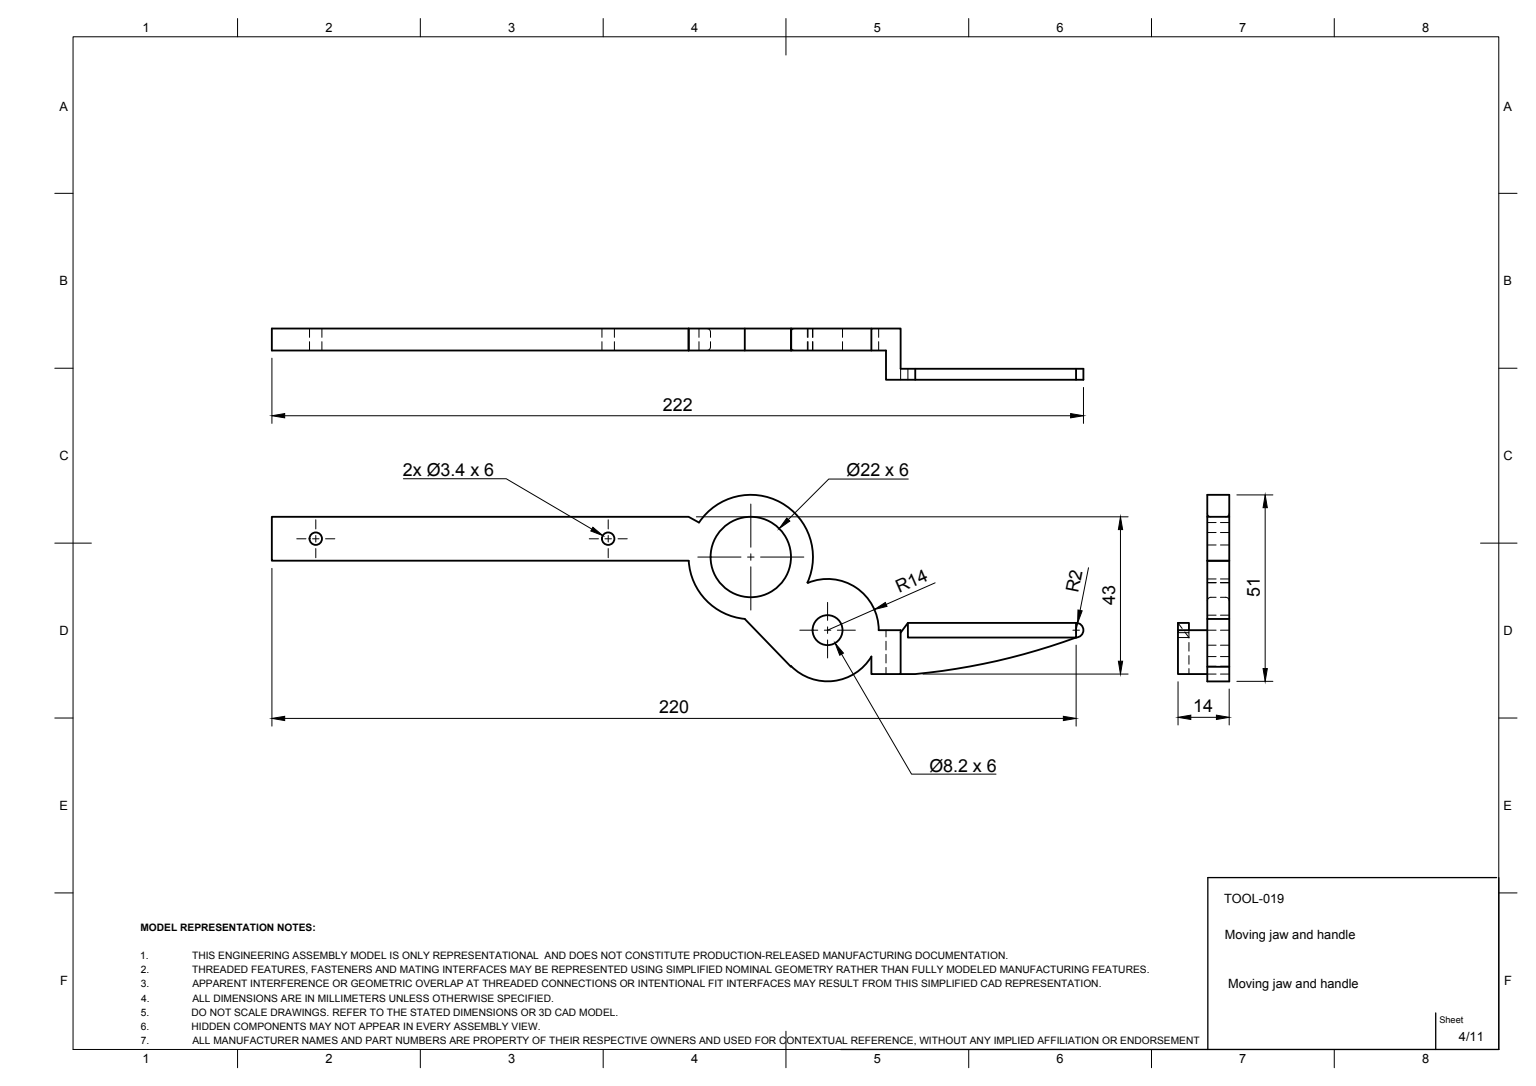
ISO-10303-21;
HEADER;
/* Generated by software containing ST-Developer
 * from STEP Tools, Inc. (www.steptools.com) 
 */

FILE_DESCRIPTION(
/* description */ (''),
/* implementation_level */ '2;1');

FILE_NAME(
/* name */ 'Moving jaw and handle.step',
/* time_stamp */ '2026-11-10T09:14:46-08:00',
/* author */ (''),
/* organization */ (''),
/* preprocessor_version */ 'ST-DEVELOPER v20.2',
/* originating_system */ 'Autodesk Translation Framework v15.17.0.0',
/* authorisation */ '');

FILE_SCHEMA (('AUTOMOTIVE_DESIGN { 1 0 10303 214 3 1 1 }'));
ENDSEC;

DATA;
#10=MECHANICAL_DESIGN_GEOMETRIC_PRESENTATION_REPRESENTATION('',(#559),#19471);
#539=SHAPE_REPRESENTATION_RELATIONSHIP('SRR','None',#19518,#549);
#549=ADVANCED_BREP_SHAPE_REPRESENTATION('',(#569),#19461);
#559=STYLED_ITEM('',(#19581),#569);
#569=MANIFOLD_SOLID_BREP('Body1',#7152);
#580=TOROIDAL_SURFACE('',#7375,1.2,0.1);
#581=TOROIDAL_SURFACE('',#7381,1.2,0.1);
#590=FACE_BOUND('',#1286,.T.);
#591=FACE_BOUND('',#1287,.T.);
#592=FACE_BOUND('',#1288,.T.);
#593=FACE_BOUND('',#1289,.T.);
#594=FACE_BOUND('',#1296,.T.);
#595=FACE_BOUND('',#1297,.T.);
#596=FACE_BOUND('',#1298,.T.);
#597=FACE_BOUND('',#1299,.T.);
#675=PLANE('',#7343);
#676=PLANE('',#7344);
#677=PLANE('',#7345);
#678=PLANE('',#7346);
#679=PLANE('',#7348);
#680=PLANE('',#7350);
#681=PLANE('',#7355);
#682=PLANE('',#7356);
#683=PLANE('',#7357);
#684=PLANE('',#7358);
#685=PLANE('',#7364);
#686=PLANE('',#7365);
#687=PLANE('',#7366);
#688=PLANE('',#7371);
#689=PLANE('',#7385);
#690=PLANE('',#7386);
#691=PLANE('',#7387);
#692=PLANE('',#7388);
#693=PLANE('',#7389);
#694=PLANE('',#7390);
#695=PLANE('',#7391);
#696=PLANE('',#7392);
#854=FACE_OUTER_BOUND('',#1271,.T.);
#855=FACE_OUTER_BOUND('',#1272,.T.);
#856=FACE_OUTER_BOUND('',#1273,.T.);
#857=FACE_OUTER_BOUND('',#1274,.T.);
#858=FACE_OUTER_BOUND('',#1275,.T.);
#859=FACE_OUTER_BOUND('',#1276,.T.);
#860=FACE_OUTER_BOUND('',#1277,.T.);
#861=FACE_OUTER_BOUND('',#1278,.T.);
#862=FACE_OUTER_BOUND('',#1279,.T.);
#863=FACE_OUTER_BOUND('',#1280,.T.);
#864=FACE_OUTER_BOUND('',#1281,.T.);
#865=FACE_OUTER_BOUND('',#1282,.T.);
#866=FACE_OUTER_BOUND('',#1283,.T.);
#867=FACE_OUTER_BOUND('',#1284,.T.);
#868=FACE_OUTER_BOUND('',#1285,.T.);
#869=FACE_OUTER_BOUND('',#1290,.T.);
#870=FACE_OUTER_BOUND('',#1291,.T.);
#871=FACE_OUTER_BOUND('',#1292,.T.);
#872=FACE_OUTER_BOUND('',#1293,.T.);
#873=FACE_OUTER_BOUND('',#1294,.T.);
#874=FACE_OUTER_BOUND('',#1295,.T.);
#875=FACE_OUTER_BOUND('',#1300,.T.);
#876=FACE_OUTER_BOUND('',#1301,.T.);
#877=FACE_OUTER_BOUND('',#1302,.T.);
#878=FACE_OUTER_BOUND('',#1303,.T.);
#879=FACE_OUTER_BOUND('',#1304,.T.);
#880=FACE_OUTER_BOUND('',#1305,.T.);
#881=FACE_OUTER_BOUND('',#1306,.T.);
#882=FACE_OUTER_BOUND('',#1307,.T.);
#883=FACE_OUTER_BOUND('',#1308,.T.);
#884=FACE_OUTER_BOUND('',#1309,.T.);
#885=FACE_OUTER_BOUND('',#1310,.T.);
#886=FACE_OUTER_BOUND('',#1311,.T.);
#887=FACE_OUTER_BOUND('',#1312,.T.);
#1271=EDGE_LOOP('',(#4721,#4722,#4723,#4724));
#1272=EDGE_LOOP('',(#4725,#4726,#4727,#4728));
#1273=EDGE_LOOP('',(#4729,#4730,#4731,#4732));
#1274=EDGE_LOOP('',(#4733,#4734,#4735));
#1275=EDGE_LOOP('',(#4736,#4737,#4738,#4739));
#1276=EDGE_LOOP('',(#4740,#4741,#4742));
#1277=EDGE_LOOP('',(#4743,#4744,#4745,#4746,#4747,#4748));
#1278=EDGE_LOOP('',(#4749,#4750));
#1279=EDGE_LOOP('',(#4751,#4752,#4753,#4754));
#1280=EDGE_LOOP('',(#4755,#4756,#4757,#4758));
#1281=EDGE_LOOP('',(#4759,#4760,#4761,#4762));
#1282=EDGE_LOOP('',(#4763,#4764,#4765,#4766,#4767,#4768,#4769,#4770));
#1283=EDGE_LOOP('',(#4771,#4772,#4773,#4774));
#1284=EDGE_LOOP('',(#4775,#4776,#4777,#4778,#4779,#4780));
#1285=EDGE_LOOP('',(#4781,#4782,#4783,#4784,#4785,#4786,#4787,#4788,#4789,
#4790,#4791,#4792,#4793,#4794,#4795,#4796));
#1286=EDGE_LOOP('',(#4797));
#1287=EDGE_LOOP('',(#4798));
#1288=EDGE_LOOP('',(#4799));
#1289=EDGE_LOOP('',(#4800));
#1290=EDGE_LOOP('',(#4801,#4802,#4803,#4804,#4805,#4806,#4807,#4808));
#1291=EDGE_LOOP('',(#4809,#4810,#4811,#4812,#4813,#4814));
#1292=EDGE_LOOP('',(#4815,#4816,#4817,#4818));
#1293=EDGE_LOOP('',(#4819,#4820,#4821,#4822));
#1294=EDGE_LOOP('',(#4823,#4824,#4825,#4826));
#1295=EDGE_LOOP('',(#4827,#4828,#4829,#4830,#4831,#4832,#4833,#4834,#4835,
#4836,#4837,#4838,#4839,#4840,#4841,#4842));
#1296=EDGE_LOOP('',(#4843));
#1297=EDGE_LOOP('',(#4844));
#1298=EDGE_LOOP('',(#4845));
#1299=EDGE_LOOP('',(#4846));
#1300=EDGE_LOOP('',(#4847,#4848,#4849,#4850));
#1301=EDGE_LOOP('',(#4851,#4852,#4853,#4854,#4855));
#1302=EDGE_LOOP('',(#4856,#4857,#4858,#4859,#4860));
#1303=EDGE_LOOP('',(#4861,#4862,#4863,#4864));
#1304=EDGE_LOOP('',(#4865,#4866,#4867,#4868));
#1305=EDGE_LOOP('',(#4869,#4870,#4871,#4872));
#1306=EDGE_LOOP('',(#4873,#4874,#4875,#4876));
#1307=EDGE_LOOP('',(#4877,#4878,#4879,#4880));
#1308=EDGE_LOOP('',(#4881,#4882,#4883,#4884));
#1309=EDGE_LOOP('',(#4885,#4886,#4887,#4888));
#1310=EDGE_LOOP('',(#4889,#4890,#4891,#4892));
#1311=EDGE_LOOP('',(#4893,#4894,#4895,#4896));
#1312=EDGE_LOOP('',(#4897,#4898,#4899,#4900));
#1774=LINE('',#9576,#2248);
#1775=LINE('',#9582,#2249);
#1776=LINE('',#9588,#2250);
#1777=LINE('',#9593,#2251);
#1778=LINE('',#9595,#2252);
#1779=LINE('',#9596,#2253);
#1780=LINE('',#9600,#2254);
#1781=LINE('',#9601,#2255);
#1782=LINE('',#9602,#2256);
#1783=LINE('',#9605,#2257);
#1784=LINE('',#9606,#2258);
#1785=LINE('',#9609,#2259);
#1786=LINE('',#9611,#2260);
#1787=LINE('',#9613,#2261);
#1788=LINE('',#9619,#2262);
#1789=LINE('',#9620,#2263);
#1790=LINE('',#9624,#2264);
#1791=LINE('',#9628,#2265);
#1792=LINE('',#9632,#2266);
#1793=LINE('',#9634,#2267);
#1794=LINE('',#9635,#2268);
#1795=LINE('',#9636,#2269);
#1796=LINE('',#9639,#2270);
#1797=LINE('',#9641,#2271);
#1798=LINE('',#9642,#2272);
#1799=LINE('',#9645,#2273);
#1800=LINE('',#9647,#2274);
#1801=LINE('',#9649,#2275);
#1802=LINE('',#9650,#2276);
#1803=LINE('',#9653,#2277);
#1804=LINE('',#9655,#2278);
#1805=LINE('',#9659,#2279);
#1806=LINE('',#9661,#2280);
#1807=LINE('',#9665,#2281);
#1808=LINE('',#9667,#2282);
#1809=LINE('',#9669,#2283);
#1810=LINE('',#9671,#2284);
#1811=LINE('',#9673,#2285);
#1812=LINE('',#9677,#2286);
#1813=LINE('',#9683,#2287);
#1814=LINE('',#9685,#2288);
#1815=LINE('',#9686,#2289);
#1816=LINE('',#9688,#2290);
#1817=LINE('',#9691,#2291);
#1818=LINE('',#9692,#2292);
#1819=LINE('',#9695,#2293);
#1820=LINE('',#9700,#2294);
#1821=LINE('',#9703,#2295);
#1822=LINE('',#9707,#2296);
#1823=LINE('',#9709,#2297);
#1824=LINE('',#9711,#2298);
#1825=LINE('',#9713,#2299);
#1826=LINE('',#9715,#2300);
#1827=LINE('',#9719,#2301);
#1828=LINE('',#9720,#2302);
#1829=LINE('',#9732,#2303);
#1830=LINE('',#9736,#2304);
#1831=LINE('',#9737,#2305);
#1832=LINE('',#9739,#2306);
#1833=LINE('',#9740,#2307);
#1834=LINE('',#9742,#2308);
#1835=LINE('',#9744,#2309);
#1836=LINE('',#9747,#2310);
#1837=LINE('',#9750,#2311);
#1838=LINE('',#9752,#2312);
#2248=VECTOR('',#8012,0.17);
#2249=VECTOR('',#8019,0.17);
#2250=VECTOR('',#8026,0.41);
#2251=VECTOR('',#8031,1.);
#2252=VECTOR('',#8032,1.);
#2253=VECTOR('',#8033,1.);
#2254=VECTOR('',#8036,1.);
#2255=VECTOR('',#8037,1.);
#2256=VECTOR('',#8038,1.);
#2257=VECTOR('',#8041,1.);
#2258=VECTOR('',#8042,1.);
#2259=VECTOR('',#8045,1.);
#2260=VECTOR('',#8046,1.);
#2261=VECTOR('',#8047,1.);
#2262=VECTOR('',#8056,1.);
#2263=VECTOR('',#8057,1.);
#2264=VECTOR('',#8062,1.);
#2265=VECTOR('',#8067,1.);
#2266=VECTOR('',#8070,1.);
#2267=VECTOR('',#8071,1.);
#2268=VECTOR('',#8072,1.);
#2269=VECTOR('',#8073,1.);
#2270=VECTOR('',#8076,1.);
#2271=VECTOR('',#8077,1.);
#2272=VECTOR('',#8078,1.);
#2273=VECTOR('',#8081,1.);
#2274=VECTOR('',#8082,1.);
#2275=VECTOR('',#8083,1.);
#2276=VECTOR('',#8084,1.);
#2277=VECTOR('',#8087,1.);
#2278=VECTOR('',#8088,1.);
#2279=VECTOR('',#8091,1.);
#2280=VECTOR('',#8092,1.);
#2281=VECTOR('',#8095,1.);
#2282=VECTOR('',#8096,1.);
#2283=VECTOR('',#8097,1.);
#2284=VECTOR('',#8098,1.);
#2285=VECTOR('',#8099,1.);
#2286=VECTOR('',#8102,1.);
#2287=VECTOR('',#8109,1.);
#2288=VECTOR('',#8110,1.);
#2289=VECTOR('',#8111,1.);
#2290=VECTOR('',#8114,1.);
#2291=VECTOR('',#8117,1.);
#2292=VECTOR('',#8118,1.);
#2293=VECTOR('',#8121,1.);
#2294=VECTOR('',#8128,1.);
#2295=VECTOR('',#8131,1.);
#2296=VECTOR('',#8134,1.);
#2297=VECTOR('',#8135,1.);
#2298=VECTOR('',#8136,1.);
#2299=VECTOR('',#8137,1.);
#2300=VECTOR('',#8138,1.);
#2301=VECTOR('',#8141,1.);
#2302=VECTOR('',#8142,1.);
#2303=VECTOR('',#8157,1.1);
#2304=VECTOR('',#8164,1.);
#2305=VECTOR('',#8165,1.);
#2306=VECTOR('',#8168,1.);
#2307=VECTOR('',#8169,1.);
#2308=VECTOR('',#8172,1.);
#2309=VECTOR('',#8175,1.);
#2310=VECTOR('',#8180,1.);
#2311=VECTOR('',#8185,1.);
#2312=VECTOR('',#8188,1.);
#2682=CIRCLE('',#7335,0.17);
#2683=CIRCLE('',#7336,0.17);
#2684=CIRCLE('',#7338,0.17);
#2685=CIRCLE('',#7339,0.17);
#2686=CIRCLE('',#7341,0.41);
#2687=CIRCLE('',#7342,0.41);
#2688=CIRCLE('',#7347,17.7082646568653);
#2689=CIRCLE('',#7349,0.2);
#2690=CIRCLE('',#7352,0.2);
#2691=CIRCLE('',#7354,17.7082646568653);
#2692=CIRCLE('',#7359,1.4);
#2693=CIRCLE('',#7360,1.7);
#2694=CIRCLE('',#7361,1.7);
#2695=CIRCLE('',#7362,1.4);
#2696=CIRCLE('',#7363,1.2);
#2697=CIRCLE('',#7368,1.4);
#2698=CIRCLE('',#7370,1.4);
#2699=CIRCLE('',#7372,1.7);
#2700=CIRCLE('',#7373,1.7);
#2701=CIRCLE('',#7374,1.2);
#2702=CIRCLE('',#7376,0.1);
#2703=CIRCLE('',#7377,1.1);
#2704=CIRCLE('',#7379,1.1);
#2705=CIRCLE('',#7380,1.1);
#2706=CIRCLE('',#7382,0.1);
#2905=VERTEX_POINT('',#9573);
#2906=VERTEX_POINT('',#9575);
#2907=VERTEX_POINT('',#9579);
#2908=VERTEX_POINT('',#9581);
#2909=VERTEX_POINT('',#9585);
#2910=VERTEX_POINT('',#9587);
#2911=VERTEX_POINT('',#9591);
#2912=VERTEX_POINT('',#9592);
#2913=VERTEX_POINT('',#9594);
#2914=VERTEX_POINT('',#9598);
#2915=VERTEX_POINT('',#9599);
#2916=VERTEX_POINT('',#9604);
#2917=VERTEX_POINT('',#9608);
#2918=VERTEX_POINT('',#9610);
#2919=VERTEX_POINT('',#9612);
#2920=VERTEX_POINT('',#9618);
#2921=VERTEX_POINT('',#9622);
#2922=VERTEX_POINT('',#9626);
#2923=VERTEX_POINT('',#9630);
#2924=VERTEX_POINT('',#9631);
#2925=VERTEX_POINT('',#9633);
#2926=VERTEX_POINT('',#9638);
#2927=VERTEX_POINT('',#9640);
#2928=VERTEX_POINT('',#9644);
#2929=VERTEX_POINT('',#9646);
#2930=VERTEX_POINT('',#9648);
#2931=VERTEX_POINT('',#9652);
#2932=VERTEX_POINT('',#9654);
#2933=VERTEX_POINT('',#9656);
#2934=VERTEX_POINT('',#9658);
#2935=VERTEX_POINT('',#9660);
#2936=VERTEX_POINT('',#9662);
#2937=VERTEX_POINT('',#9664);
#2938=VERTEX_POINT('',#9666);
#2939=VERTEX_POINT('',#9668);
#2940=VERTEX_POINT('',#9670);
#2941=VERTEX_POINT('',#9672);
#2942=VERTEX_POINT('',#9674);
#2943=VERTEX_POINT('',#9676);
#2944=VERTEX_POINT('',#9679);
#2945=VERTEX_POINT('',#9682);
#2946=VERTEX_POINT('',#9684);
#2947=VERTEX_POINT('',#9690);
#2948=VERTEX_POINT('',#9694);
#2949=VERTEX_POINT('',#9698);
#2950=VERTEX_POINT('',#9702);
#2951=VERTEX_POINT('',#9704);
#2952=VERTEX_POINT('',#9706);
#2953=VERTEX_POINT('',#9708);
#2954=VERTEX_POINT('',#9710);
#2955=VERTEX_POINT('',#9712);
#2956=VERTEX_POINT('',#9714);
#2957=VERTEX_POINT('',#9716);
#2958=VERTEX_POINT('',#9718);
#2959=VERTEX_POINT('',#9721);
#2960=VERTEX_POINT('',#9724);
#2961=VERTEX_POINT('',#9728);
#2962=VERTEX_POINT('',#9729);
#3601=EDGE_CURVE('',#2905,#2905,#2682,.T.);
#3602=EDGE_CURVE('',#2905,#2906,#1774,.T.);
#3603=EDGE_CURVE('',#2906,#2906,#2683,.T.);
#3604=EDGE_CURVE('',#2907,#2907,#2684,.T.);
#3605=EDGE_CURVE('',#2907,#2908,#1775,.T.);
#3606=EDGE_CURVE('',#2908,#2908,#2685,.T.);
#3607=EDGE_CURVE('',#2909,#2909,#2686,.T.);
#3608=EDGE_CURVE('',#2909,#2910,#1776,.T.);
#3609=EDGE_CURVE('',#2910,#2910,#2687,.T.);
#3610=EDGE_CURVE('',#2911,#2912,#1777,.T.);
#3611=EDGE_CURVE('',#2913,#2911,#1778,.T.);
#3612=EDGE_CURVE('',#2913,#2912,#1779,.T.);
#3613=EDGE_CURVE('',#2914,#2915,#1780,.T.);
#3614=EDGE_CURVE('',#2913,#2914,#1781,.T.);
#3615=EDGE_CURVE('',#2915,#2911,#1782,.T.);
#3616=EDGE_CURVE('',#2916,#2915,#1783,.T.);
#3617=EDGE_CURVE('',#2914,#2916,#1784,.T.);
#3618=EDGE_CURVE('',#2912,#2917,#1785,.T.);
#3619=EDGE_CURVE('',#2918,#2917,#1786,.T.);
#3620=EDGE_CURVE('',#2918,#2919,#1787,.T.);
#3621=EDGE_CURVE('',#2919,#2915,#2688,.T.);
#3622=EDGE_CURVE('',#2915,#2916,#2689,.T.);
#3623=EDGE_CURVE('',#2917,#2920,#1788,.T.);
#3624=EDGE_CURVE('',#2920,#2913,#1789,.T.);
#3625=EDGE_CURVE('',#2921,#2914,#2690,.T.);
#3626=EDGE_CURVE('',#2921,#2915,#1790,.T.);
#3627=EDGE_CURVE('',#2922,#2921,#2691,.T.);
#3628=EDGE_CURVE('',#2922,#2919,#1791,.T.);
#3629=EDGE_CURVE('',#2923,#2924,#1792,.T.);
#3630=EDGE_CURVE('',#2924,#2925,#1793,.T.);
#3631=EDGE_CURVE('',#2925,#2920,#1794,.T.);
#3632=EDGE_CURVE('',#2922,#2923,#1795,.T.);
#3633=EDGE_CURVE('',#2923,#2926,#1796,.T.);
#3634=EDGE_CURVE('',#2927,#2926,#1797,.T.);
#3635=EDGE_CURVE('',#2924,#2927,#1798,.T.);
#3636=EDGE_CURVE('',#2928,#2927,#1799,.T.);
#3637=EDGE_CURVE('',#2929,#2928,#1800,.T.);
#3638=EDGE_CURVE('',#2930,#2929,#1801,.T.);
#3639=EDGE_CURVE('',#2925,#2930,#1802,.T.);
#3640=EDGE_CURVE('',#2926,#2931,#1803,.T.);
#3641=EDGE_CURVE('',#2931,#2932,#1804,.T.);
#3642=EDGE_CURVE('',#2933,#2932,#2692,.T.);
#3643=EDGE_CURVE('',#2934,#2933,#1805,.T.);
#3644=EDGE_CURVE('',#2935,#2934,#1806,.T.);
#3645=EDGE_CURVE('',#2936,#2935,#2693,.T.);
#3646=EDGE_CURVE('',#2937,#2936,#1807,.T.);
#3647=EDGE_CURVE('',#2938,#2937,#1808,.T.);
#3648=EDGE_CURVE('',#2939,#2938,#1809,.T.);
#3649=EDGE_CURVE('',#2940,#2939,#1810,.T.);
#3650=EDGE_CURVE('',#2941,#2940,#1811,.T.);
#3651=EDGE_CURVE('',#2942,#2941,#2694,.T.);
#3652=EDGE_CURVE('',#2943,#2942,#1812,.T.);
#3653=EDGE_CURVE('',#2928,#2943,#2695,.T.);
#3654=EDGE_CURVE('',#2944,#2944,#2696,.T.);
#3655=EDGE_CURVE('',#2918,#2945,#1813,.T.);
#3656=EDGE_CURVE('',#2946,#2945,#1814,.T.);
#3657=EDGE_CURVE('',#2931,#2946,#1815,.T.);
#3658=EDGE_CURVE('',#2945,#2930,#1816,.T.);
#3659=EDGE_CURVE('',#2932,#2947,#1817,.T.);
#3660=EDGE_CURVE('',#2947,#2946,#1818,.T.);
#3661=EDGE_CURVE('',#2943,#2948,#1819,.T.);
#3662=EDGE_CURVE('',#2929,#2948,#2697,.T.);
#3663=EDGE_CURVE('',#2949,#2947,#2698,.T.);
#3664=EDGE_CURVE('',#2949,#2933,#1820,.T.);
#3665=EDGE_CURVE('',#2948,#2950,#1821,.T.);
#3666=EDGE_CURVE('',#2950,#2951,#2699,.T.);
#3667=EDGE_CURVE('',#2951,#2952,#1822,.T.);
#3668=EDGE_CURVE('',#2952,#2953,#1823,.T.);
#3669=EDGE_CURVE('',#2953,#2954,#1824,.T.);
#3670=EDGE_CURVE('',#2954,#2955,#1825,.T.);
#3671=EDGE_CURVE('',#2955,#2956,#1826,.T.);
#3672=EDGE_CURVE('',#2956,#2957,#2700,.T.);
#3673=EDGE_CURVE('',#2957,#2958,#1827,.T.);
#3674=EDGE_CURVE('',#2958,#2949,#1828,.T.);
#3675=EDGE_CURVE('',#2959,#2959,#2701,.T.);
#3676=EDGE_CURVE('',#2944,#2960,#2702,.T.);
#3677=EDGE_CURVE('',#2960,#2960,#2703,.T.);
#3678=EDGE_CURVE('',#2961,#2962,#2704,.T.);
#3679=EDGE_CURVE('',#2962,#2961,#2705,.T.);
#3680=EDGE_CURVE('',#2962,#2960,#1829,.T.);
#3681=EDGE_CURVE('',#2959,#2961,#2706,.T.);
#3682=EDGE_CURVE('',#2957,#2935,#1830,.T.);
#3683=EDGE_CURVE('',#2936,#2956,#1831,.T.);
#3684=EDGE_CURVE('',#2942,#2950,#1832,.T.);
#3685=EDGE_CURVE('',#2951,#2941,#1833,.T.);
#3686=EDGE_CURVE('',#2940,#2952,#1834,.T.);
#3687=EDGE_CURVE('',#2937,#2955,#1835,.T.);
#3688=EDGE_CURVE('',#2934,#2958,#1836,.T.);
#3689=EDGE_CURVE('',#2938,#2954,#1837,.T.);
#3690=EDGE_CURVE('',#2939,#2953,#1838,.T.);
#4721=ORIENTED_EDGE('',*,*,#3601,.F.);
#4722=ORIENTED_EDGE('',*,*,#3602,.T.);
#4723=ORIENTED_EDGE('',*,*,#3603,.F.);
#4724=ORIENTED_EDGE('',*,*,#3602,.F.);
#4725=ORIENTED_EDGE('',*,*,#3604,.F.);
#4726=ORIENTED_EDGE('',*,*,#3605,.T.);
#4727=ORIENTED_EDGE('',*,*,#3606,.F.);
#4728=ORIENTED_EDGE('',*,*,#3605,.F.);
#4729=ORIENTED_EDGE('',*,*,#3607,.F.);
#4730=ORIENTED_EDGE('',*,*,#3608,.T.);
#4731=ORIENTED_EDGE('',*,*,#3609,.F.);
#4732=ORIENTED_EDGE('',*,*,#3608,.F.);
#4733=ORIENTED_EDGE('',*,*,#3610,.F.);
#4734=ORIENTED_EDGE('',*,*,#3611,.F.);
#4735=ORIENTED_EDGE('',*,*,#3612,.T.);
#4736=ORIENTED_EDGE('',*,*,#3613,.F.);
#4737=ORIENTED_EDGE('',*,*,#3614,.F.);
#4738=ORIENTED_EDGE('',*,*,#3611,.T.);
#4739=ORIENTED_EDGE('',*,*,#3615,.F.);
#4740=ORIENTED_EDGE('',*,*,#3616,.F.);
#4741=ORIENTED_EDGE('',*,*,#3617,.F.);
#4742=ORIENTED_EDGE('',*,*,#3613,.T.);
#4743=ORIENTED_EDGE('',*,*,#3615,.T.);
#4744=ORIENTED_EDGE('',*,*,#3610,.T.);
#4745=ORIENTED_EDGE('',*,*,#3618,.T.);
#4746=ORIENTED_EDGE('',*,*,#3619,.F.);
#4747=ORIENTED_EDGE('',*,*,#3620,.T.);
#4748=ORIENTED_EDGE('',*,*,#3621,.T.);
#4749=ORIENTED_EDGE('',*,*,#3616,.T.);
#4750=ORIENTED_EDGE('',*,*,#3622,.T.);
#4751=ORIENTED_EDGE('',*,*,#3623,.F.);
#4752=ORIENTED_EDGE('',*,*,#3618,.F.);
#4753=ORIENTED_EDGE('',*,*,#3612,.F.);
#4754=ORIENTED_EDGE('',*,*,#3624,.F.);
#4755=ORIENTED_EDGE('',*,*,#3625,.T.);
#4756=ORIENTED_EDGE('',*,*,#3617,.T.);
#4757=ORIENTED_EDGE('',*,*,#3622,.F.);
#4758=ORIENTED_EDGE('',*,*,#3626,.F.);
#4759=ORIENTED_EDGE('',*,*,#3627,.T.);
#4760=ORIENTED_EDGE('',*,*,#3626,.T.);
#4761=ORIENTED_EDGE('',*,*,#3621,.F.);
#4762=ORIENTED_EDGE('',*,*,#3628,.F.);
#4763=ORIENTED_EDGE('',*,*,#3629,.T.);
#4764=ORIENTED_EDGE('',*,*,#3630,.T.);
#4765=ORIENTED_EDGE('',*,*,#3631,.T.);
#4766=ORIENTED_EDGE('',*,*,#3624,.T.);
#4767=ORIENTED_EDGE('',*,*,#3614,.T.);
#4768=ORIENTED_EDGE('',*,*,#3625,.F.);
#4769=ORIENTED_EDGE('',*,*,#3627,.F.);
#4770=ORIENTED_EDGE('',*,*,#3632,.T.);
#4771=ORIENTED_EDGE('',*,*,#3629,.F.);
#4772=ORIENTED_EDGE('',*,*,#3633,.T.);
#4773=ORIENTED_EDGE('',*,*,#3634,.F.);
#4774=ORIENTED_EDGE('',*,*,#3635,.F.);
#4775=ORIENTED_EDGE('',*,*,#3636,.F.);
#4776=ORIENTED_EDGE('',*,*,#3637,.F.);
#4777=ORIENTED_EDGE('',*,*,#3638,.F.);
#4778=ORIENTED_EDGE('',*,*,#3639,.F.);
#4779=ORIENTED_EDGE('',*,*,#3630,.F.);
#4780=ORIENTED_EDGE('',*,*,#3635,.T.);
#4781=ORIENTED_EDGE('',*,*,#3634,.T.);
#4782=ORIENTED_EDGE('',*,*,#3640,.T.);
#4783=ORIENTED_EDGE('',*,*,#3641,.T.);
#4784=ORIENTED_EDGE('',*,*,#3642,.F.);
#4785=ORIENTED_EDGE('',*,*,#3643,.F.);
#4786=ORIENTED_EDGE('',*,*,#3644,.F.);
#4787=ORIENTED_EDGE('',*,*,#3645,.F.);
#4788=ORIENTED_EDGE('',*,*,#3646,.F.);
#4789=ORIENTED_EDGE('',*,*,#3647,.F.);
#4790=ORIENTED_EDGE('',*,*,#3648,.F.);
#4791=ORIENTED_EDGE('',*,*,#3649,.F.);
#4792=ORIENTED_EDGE('',*,*,#3650,.F.);
#4793=ORIENTED_EDGE('',*,*,#3651,.F.);
#4794=ORIENTED_EDGE('',*,*,#3652,.F.);
#4795=ORIENTED_EDGE('',*,*,#3653,.F.);
#4796=ORIENTED_EDGE('',*,*,#3636,.T.);
#4797=ORIENTED_EDGE('',*,*,#3603,.T.);
#4798=ORIENTED_EDGE('',*,*,#3606,.T.);
#4799=ORIENTED_EDGE('',*,*,#3609,.T.);
#4800=ORIENTED_EDGE('',*,*,#3654,.F.);
#4801=ORIENTED_EDGE('',*,*,#3655,.T.);
#4802=ORIENTED_EDGE('',*,*,#3656,.F.);
#4803=ORIENTED_EDGE('',*,*,#3657,.F.);
#4804=ORIENTED_EDGE('',*,*,#3640,.F.);
#4805=ORIENTED_EDGE('',*,*,#3633,.F.);
#4806=ORIENTED_EDGE('',*,*,#3632,.F.);
#4807=ORIENTED_EDGE('',*,*,#3628,.T.);
#4808=ORIENTED_EDGE('',*,*,#3620,.F.);
#4809=ORIENTED_EDGE('',*,*,#3623,.T.);
#4810=ORIENTED_EDGE('',*,*,#3631,.F.);
#4811=ORIENTED_EDGE('',*,*,#3639,.T.);
#4812=ORIENTED_EDGE('',*,*,#3658,.F.);
#4813=ORIENTED_EDGE('',*,*,#3655,.F.);
#4814=ORIENTED_EDGE('',*,*,#3619,.T.);
#4815=ORIENTED_EDGE('',*,*,#3659,.F.);
#4816=ORIENTED_EDGE('',*,*,#3641,.F.);
#4817=ORIENTED_EDGE('',*,*,#3657,.T.);
#4818=ORIENTED_EDGE('',*,*,#3660,.F.);
#4819=ORIENTED_EDGE('',*,*,#3637,.T.);
#4820=ORIENTED_EDGE('',*,*,#3653,.T.);
#4821=ORIENTED_EDGE('',*,*,#3661,.T.);
#4822=ORIENTED_EDGE('',*,*,#3662,.F.);
#4823=ORIENTED_EDGE('',*,*,#3659,.T.);
#4824=ORIENTED_EDGE('',*,*,#3663,.F.);
#4825=ORIENTED_EDGE('',*,*,#3664,.T.);
#4826=ORIENTED_EDGE('',*,*,#3642,.T.);
#4827=ORIENTED_EDGE('',*,*,#3638,.T.);
#4828=ORIENTED_EDGE('',*,*,#3662,.T.);
#4829=ORIENTED_EDGE('',*,*,#3665,.T.);
#4830=ORIENTED_EDGE('',*,*,#3666,.T.);
#4831=ORIENTED_EDGE('',*,*,#3667,.T.);
#4832=ORIENTED_EDGE('',*,*,#3668,.T.);
#4833=ORIENTED_EDGE('',*,*,#3669,.T.);
#4834=ORIENTED_EDGE('',*,*,#3670,.T.);
#4835=ORIENTED_EDGE('',*,*,#3671,.T.);
#4836=ORIENTED_EDGE('',*,*,#3672,.T.);
#4837=ORIENTED_EDGE('',*,*,#3673,.T.);
#4838=ORIENTED_EDGE('',*,*,#3674,.T.);
#4839=ORIENTED_EDGE('',*,*,#3663,.T.);
#4840=ORIENTED_EDGE('',*,*,#3660,.T.);
#4841=ORIENTED_EDGE('',*,*,#3656,.T.);
#4842=ORIENTED_EDGE('',*,*,#3658,.T.);
#4843=ORIENTED_EDGE('',*,*,#3601,.T.);
#4844=ORIENTED_EDGE('',*,*,#3604,.T.);
#4845=ORIENTED_EDGE('',*,*,#3607,.T.);
#4846=ORIENTED_EDGE('',*,*,#3675,.F.);
#4847=ORIENTED_EDGE('',*,*,#3654,.T.);
#4848=ORIENTED_EDGE('',*,*,#3676,.T.);
#4849=ORIENTED_EDGE('',*,*,#3677,.T.);
#4850=ORIENTED_EDGE('',*,*,#3676,.F.);
#4851=ORIENTED_EDGE('',*,*,#3678,.F.);
#4852=ORIENTED_EDGE('',*,*,#3679,.F.);
#4853=ORIENTED_EDGE('',*,*,#3680,.T.);
#4854=ORIENTED_EDGE('',*,*,#3677,.F.);
#4855=ORIENTED_EDGE('',*,*,#3680,.F.);
#4856=ORIENTED_EDGE('',*,*,#3675,.T.);
#4857=ORIENTED_EDGE('',*,*,#3681,.T.);
#4858=ORIENTED_EDGE('',*,*,#3678,.T.);
#4859=ORIENTED_EDGE('',*,*,#3679,.T.);
#4860=ORIENTED_EDGE('',*,*,#3681,.F.);
#4861=ORIENTED_EDGE('',*,*,#3682,.F.);
#4862=ORIENTED_EDGE('',*,*,#3672,.F.);
#4863=ORIENTED_EDGE('',*,*,#3683,.F.);
#4864=ORIENTED_EDGE('',*,*,#3645,.T.);
#4865=ORIENTED_EDGE('',*,*,#3684,.F.);
#4866=ORIENTED_EDGE('',*,*,#3651,.T.);
#4867=ORIENTED_EDGE('',*,*,#3685,.F.);
#4868=ORIENTED_EDGE('',*,*,#3666,.F.);
#4869=ORIENTED_EDGE('',*,*,#3685,.T.);
#4870=ORIENTED_EDGE('',*,*,#3650,.T.);
#4871=ORIENTED_EDGE('',*,*,#3686,.T.);
#4872=ORIENTED_EDGE('',*,*,#3667,.F.);
#4873=ORIENTED_EDGE('',*,*,#3683,.T.);
#4874=ORIENTED_EDGE('',*,*,#3671,.F.);
#4875=ORIENTED_EDGE('',*,*,#3687,.F.);
#4876=ORIENTED_EDGE('',*,*,#3646,.T.);
#4877=ORIENTED_EDGE('',*,*,#3684,.T.);
#4878=ORIENTED_EDGE('',*,*,#3665,.F.);
#4879=ORIENTED_EDGE('',*,*,#3661,.F.);
#4880=ORIENTED_EDGE('',*,*,#3652,.T.);
#4881=ORIENTED_EDGE('',*,*,#3664,.F.);
#4882=ORIENTED_EDGE('',*,*,#3674,.F.);
#4883=ORIENTED_EDGE('',*,*,#3688,.F.);
#4884=ORIENTED_EDGE('',*,*,#3643,.T.);
#4885=ORIENTED_EDGE('',*,*,#3682,.T.);
#4886=ORIENTED_EDGE('',*,*,#3644,.T.);
#4887=ORIENTED_EDGE('',*,*,#3688,.T.);
#4888=ORIENTED_EDGE('',*,*,#3673,.F.);
#4889=ORIENTED_EDGE('',*,*,#3647,.T.);
#4890=ORIENTED_EDGE('',*,*,#3687,.T.);
#4891=ORIENTED_EDGE('',*,*,#3670,.F.);
#4892=ORIENTED_EDGE('',*,*,#3689,.F.);
#4893=ORIENTED_EDGE('',*,*,#3648,.T.);
#4894=ORIENTED_EDGE('',*,*,#3689,.T.);
#4895=ORIENTED_EDGE('',*,*,#3669,.F.);
#4896=ORIENTED_EDGE('',*,*,#3690,.F.);
#4897=ORIENTED_EDGE('',*,*,#3649,.T.);
#4898=ORIENTED_EDGE('',*,*,#3690,.T.);
#4899=ORIENTED_EDGE('',*,*,#3668,.F.);
#4900=ORIENTED_EDGE('',*,*,#3686,.F.);
#6611=CYLINDRICAL_SURFACE('',#7334,0.17);
#6612=CYLINDRICAL_SURFACE('',#7337,0.17);
#6613=CYLINDRICAL_SURFACE('',#7340,0.41);
#6614=CYLINDRICAL_SURFACE('',#7351,0.2);
#6615=CYLINDRICAL_SURFACE('',#7353,17.7082646568653);
#6616=CYLINDRICAL_SURFACE('',#7367,1.4);
#6617=CYLINDRICAL_SURFACE('',#7369,1.4);
#6618=CYLINDRICAL_SURFACE('',#7378,1.1);
#6619=CYLINDRICAL_SURFACE('',#7383,1.7);
#6620=CYLINDRICAL_SURFACE('',#7384,1.7);
#6776=ADVANCED_FACE('',(#854),#6611,.F.);
#6777=ADVANCED_FACE('',(#855),#6612,.F.);
#6778=ADVANCED_FACE('',(#856),#6613,.F.);
#6779=ADVANCED_FACE('',(#857),#675,.F.);
#6780=ADVANCED_FACE('',(#858),#676,.F.);
#6781=ADVANCED_FACE('',(#859),#677,.T.);
#6782=ADVANCED_FACE('',(#860),#678,.T.);
#6783=ADVANCED_FACE('',(#861),#679,.T.);
#6784=ADVANCED_FACE('',(#862),#680,.T.);
#6785=ADVANCED_FACE('',(#863),#6614,.T.);
#6786=ADVANCED_FACE('',(#864),#6615,.T.);
#6787=ADVANCED_FACE('',(#865),#681,.F.);
#6788=ADVANCED_FACE('',(#866),#682,.T.);
#6789=ADVANCED_FACE('',(#867),#683,.T.);
#6790=ADVANCED_FACE('',(#868,#590,#591,#592,#593),#684,.F.);
#6791=ADVANCED_FACE('',(#869),#685,.T.);
#6792=ADVANCED_FACE('',(#870),#686,.T.);
#6793=ADVANCED_FACE('',(#871),#687,.T.);
#6794=ADVANCED_FACE('',(#872),#6616,.T.);
#6795=ADVANCED_FACE('',(#873),#6617,.T.);
#6796=ADVANCED_FACE('',(#874,#594,#595,#596,#597),#688,.T.);
#6797=ADVANCED_FACE('',(#875),#580,.T.);
#6798=ADVANCED_FACE('',(#876),#6618,.F.);
#6799=ADVANCED_FACE('',(#877),#581,.T.);
#6800=ADVANCED_FACE('',(#878),#6619,.T.);
#6801=ADVANCED_FACE('',(#879),#6620,.T.);
#6802=ADVANCED_FACE('',(#880),#689,.T.);
#6803=ADVANCED_FACE('',(#881),#690,.T.);
#6804=ADVANCED_FACE('',(#882),#691,.T.);
#6805=ADVANCED_FACE('',(#883),#692,.T.);
#6806=ADVANCED_FACE('',(#884),#693,.T.);
#6807=ADVANCED_FACE('',(#885),#694,.T.);
#6808=ADVANCED_FACE('',(#886),#695,.T.);
#6809=ADVANCED_FACE('',(#887),#696,.T.);
#7152=CLOSED_SHELL('',(#6776,#6777,#6778,#6779,#6780,#6781,#6782,#6783,
#6784,#6785,#6786,#6787,#6788,#6789,#6790,#6791,#6792,#6793,#6794,#6795,
#6796,#6797,#6798,#6799,#6800,#6801,#6802,#6803,#6804,#6805,#6806,#6807,
#6808,#6809));
#7333=AXIS2_PLACEMENT_3D('',#9571,#8006,#8007);
#7334=AXIS2_PLACEMENT_3D('',#9572,#8008,#8009);
#7335=AXIS2_PLACEMENT_3D('',#9574,#8010,#8011);
#7336=AXIS2_PLACEMENT_3D('',#9577,#8013,#8014);
#7337=AXIS2_PLACEMENT_3D('',#9578,#8015,#8016);
#7338=AXIS2_PLACEMENT_3D('',#9580,#8017,#8018);
#7339=AXIS2_PLACEMENT_3D('',#9583,#8020,#8021);
#7340=AXIS2_PLACEMENT_3D('',#9584,#8022,#8023);
#7341=AXIS2_PLACEMENT_3D('',#9586,#8024,#8025);
#7342=AXIS2_PLACEMENT_3D('',#9589,#8027,#8028);
#7343=AXIS2_PLACEMENT_3D('',#9590,#8029,#8030);
#7344=AXIS2_PLACEMENT_3D('',#9597,#8034,#8035);
#7345=AXIS2_PLACEMENT_3D('',#9603,#8039,#8040);
#7346=AXIS2_PLACEMENT_3D('',#9607,#8043,#8044);
#7347=AXIS2_PLACEMENT_3D('',#9614,#8048,#8049);
#7348=AXIS2_PLACEMENT_3D('',#9615,#8050,#8051);
#7349=AXIS2_PLACEMENT_3D('',#9616,#8052,#8053);
#7350=AXIS2_PLACEMENT_3D('',#9617,#8054,#8055);
#7351=AXIS2_PLACEMENT_3D('',#9621,#8058,#8059);
#7352=AXIS2_PLACEMENT_3D('',#9623,#8060,#8061);
#7353=AXIS2_PLACEMENT_3D('',#9625,#8063,#8064);
#7354=AXIS2_PLACEMENT_3D('',#9627,#8065,#8066);
#7355=AXIS2_PLACEMENT_3D('',#9629,#8068,#8069);
#7356=AXIS2_PLACEMENT_3D('',#9637,#8074,#8075);
#7357=AXIS2_PLACEMENT_3D('',#9643,#8079,#8080);
#7358=AXIS2_PLACEMENT_3D('',#9651,#8085,#8086);
#7359=AXIS2_PLACEMENT_3D('',#9657,#8089,#8090);
#7360=AXIS2_PLACEMENT_3D('',#9663,#8093,#8094);
#7361=AXIS2_PLACEMENT_3D('',#9675,#8100,#8101);
#7362=AXIS2_PLACEMENT_3D('',#9678,#8103,#8104);
#7363=AXIS2_PLACEMENT_3D('',#9680,#8105,#8106);
#7364=AXIS2_PLACEMENT_3D('',#9681,#8107,#8108);
#7365=AXIS2_PLACEMENT_3D('',#9687,#8112,#8113);
#7366=AXIS2_PLACEMENT_3D('',#9689,#8115,#8116);
#7367=AXIS2_PLACEMENT_3D('',#9693,#8119,#8120);
#7368=AXIS2_PLACEMENT_3D('',#9696,#8122,#8123);
#7369=AXIS2_PLACEMENT_3D('',#9697,#8124,#8125);
#7370=AXIS2_PLACEMENT_3D('',#9699,#8126,#8127);
#7371=AXIS2_PLACEMENT_3D('',#9701,#8129,#8130);
#7372=AXIS2_PLACEMENT_3D('',#9705,#8132,#8133);
#7373=AXIS2_PLACEMENT_3D('',#9717,#8139,#8140);
#7374=AXIS2_PLACEMENT_3D('',#9722,#8143,#8144);
#7375=AXIS2_PLACEMENT_3D('',#9723,#8145,#8146);
#7376=AXIS2_PLACEMENT_3D('',#9725,#8147,#8148);
#7377=AXIS2_PLACEMENT_3D('',#9726,#8149,#8150);
#7378=AXIS2_PLACEMENT_3D('',#9727,#8151,#8152);
#7379=AXIS2_PLACEMENT_3D('',#9730,#8153,#8154);
#7380=AXIS2_PLACEMENT_3D('',#9731,#8155,#8156);
#7381=AXIS2_PLACEMENT_3D('',#9733,#8158,#8159);
#7382=AXIS2_PLACEMENT_3D('',#9734,#8160,#8161);
#7383=AXIS2_PLACEMENT_3D('',#9735,#8162,#8163);
#7384=AXIS2_PLACEMENT_3D('',#9738,#8166,#8167);
#7385=AXIS2_PLACEMENT_3D('',#9741,#8170,#8171);
#7386=AXIS2_PLACEMENT_3D('',#9743,#8173,#8174);
#7387=AXIS2_PLACEMENT_3D('',#9745,#8176,#8177);
#7388=AXIS2_PLACEMENT_3D('',#9746,#8178,#8179);
#7389=AXIS2_PLACEMENT_3D('',#9748,#8181,#8182);
#7390=AXIS2_PLACEMENT_3D('',#9749,#8183,#8184);
#7391=AXIS2_PLACEMENT_3D('',#9751,#8186,#8187);
#7392=AXIS2_PLACEMENT_3D('',#9753,#8189,#8190);
#8006=DIRECTION('axis',(0.,0.,1.));
#8007=DIRECTION('refdir',(1.,0.,0.));
#8008=DIRECTION('center_axis',(0.,0.,-1.));
#8009=DIRECTION('ref_axis',(1.,0.,0.));
#8010=DIRECTION('center_axis',(0.,0.,-1.));
#8011=DIRECTION('ref_axis',(1.,0.,0.));
#8012=DIRECTION('',(0.,0.,-1.));
#8013=DIRECTION('center_axis',(0.,0.,1.));
#8014=DIRECTION('ref_axis',(1.,0.,0.));
#8015=DIRECTION('center_axis',(0.,0.,-1.));
#8016=DIRECTION('ref_axis',(1.,0.,0.));
#8017=DIRECTION('center_axis',(0.,0.,-1.));
#8018=DIRECTION('ref_axis',(1.,0.,0.));
#8019=DIRECTION('',(0.,0.,-1.));
#8020=DIRECTION('center_axis',(0.,0.,1.));
#8021=DIRECTION('ref_axis',(1.,0.,0.));
#8022=DIRECTION('center_axis',(0.,0.,-1.));
#8023=DIRECTION('ref_axis',(1.,0.,0.));
#8024=DIRECTION('center_axis',(0.,0.,-1.));
#8025=DIRECTION('ref_axis',(1.,0.,0.));
#8026=DIRECTION('',(0.,0.,-1.));
#8027=DIRECTION('center_axis',(0.,0.,1.));
#8028=DIRECTION('ref_axis',(1.,0.,0.));
#8029=DIRECTION('center_axis',(1.,0.,0.));
#8030=DIRECTION('ref_axis',(0.,0.,-1.));
#8031=DIRECTION('',(0.,-1.,0.));
#8032=DIRECTION('',(0.,0.8,0.6));
#8033=DIRECTION('',(0.,0.,1.));
#8034=DIRECTION('center_axis',(0.,0.6,-0.8));
#8035=DIRECTION('ref_axis',(0.,0.8,0.6));
#8036=DIRECTION('',(0.,0.8,0.6));
#8037=DIRECTION('',(-1.,0.,0.));
#8038=DIRECTION('',(1.,0.,0.));
#8039=DIRECTION('center_axis',(1.,0.,0.));
#8040=DIRECTION('ref_axis',(0.,2.22044604925031E-16,1.));
#8041=DIRECTION('',(0.,1.,0.));
#8042=DIRECTION('',(0.,0.,1.));
#8043=DIRECTION('center_axis',(0.,0.,1.));
#8044=DIRECTION('ref_axis',(1.,0.,0.));
#8045=DIRECTION('',(0.6,0.8,0.));
#8046=DIRECTION('',(0.,-1.,0.));
#8047=DIRECTION('',(-1.,0.,0.));
#8048=DIRECTION('center_axis',(0.,0.,1.));
#8049=DIRECTION('ref_axis',(-0.0955793180441842,0.995421817101779,0.));
#8050=DIRECTION('center_axis',(0.,0.,1.));
#8051=DIRECTION('ref_axis',(1.,0.,0.));
#8052=DIRECTION('center_axis',(0.,0.,1.));
#8053=DIRECTION('ref_axis',(4.44089209850063E-15,1.,0.));
#8054=DIRECTION('center_axis',(0.8,-0.6,0.));
#8055=DIRECTION('ref_axis',(0.6,0.8,0.));
#8056=DIRECTION('',(0.,0.,-1.));
#8057=DIRECTION('',(-0.6,-0.8,0.));
#8058=DIRECTION('center_axis',(0.,0.,1.));
#8059=DIRECTION('ref_axis',(4.44089209850063E-15,1.,0.));
#8060=DIRECTION('center_axis',(0.,0.,1.));
#8061=DIRECTION('ref_axis',(4.44089209850063E-15,1.,0.));
#8062=DIRECTION('',(0.,0.,1.));
#8063=DIRECTION('center_axis',(0.,0.,1.));
#8064=DIRECTION('ref_axis',(-0.0955793180441842,0.995421817101779,0.));
#8065=DIRECTION('center_axis',(0.,0.,1.));
#8066=DIRECTION('ref_axis',(-0.0955793180441842,0.995421817101779,0.));
#8067=DIRECTION('',(0.,0.,1.));
#8068=DIRECTION('center_axis',(0.,0.,1.));
#8069=DIRECTION('ref_axis',(1.,0.,0.));
#8070=DIRECTION('',(0.,-1.,0.));
#8071=DIRECTION('',(-1.,0.,0.));
#8072=DIRECTION('',(0.,1.,0.));
#8073=DIRECTION('',(1.,0.,0.));
#8074=DIRECTION('center_axis',(1.,0.,0.));
#8075=DIRECTION('ref_axis',(0.,1.,0.));
#8076=DIRECTION('',(0.,0.,1.));
#8077=DIRECTION('',(0.,1.,0.));
#8078=DIRECTION('',(0.,0.,1.));
#8079=DIRECTION('center_axis',(0.,-1.,0.));
#8080=DIRECTION('ref_axis',(1.,0.,0.));
#8081=DIRECTION('',(-1.,0.,0.));
#8082=DIRECTION('',(0.,0.,-1.));
#8083=DIRECTION('',(1.,0.,0.));
#8084=DIRECTION('',(0.,0.,1.));
#8085=DIRECTION('center_axis',(0.,0.,1.));
#8086=DIRECTION('ref_axis',(1.,0.,0.));
#8087=DIRECTION('',(1.,0.,0.));
#8088=DIRECTION('',(0.,-1.,0.));
#8089=DIRECTION('center_axis',(0.,0.,1.));
#8090=DIRECTION('ref_axis',(1.,0.,0.));
#8091=DIRECTION('',(-0.447213595499958,-0.894427190999916,0.));
#8092=DIRECTION('',(-0.694594513699567,0.719401460617409,0.));
#8093=DIRECTION('center_axis',(0.,0.,1.));
#8094=DIRECTION('ref_axis',(1.,0.,0.));
#8095=DIRECTION('',(-0.694594513699567,0.719401460617409,0.));
#8096=DIRECTION('',(-1.,0.,0.));
#8097=DIRECTION('',(0.,1.,0.));
#8098=DIRECTION('',(1.,0.,0.));
#8099=DIRECTION('',(0.87524153543927,-0.483686111690123,0.));
#8100=DIRECTION('center_axis',(0.,0.,1.));
#8101=DIRECTION('ref_axis',(1.,0.,0.));
#8102=DIRECTION('',(0.87524153543927,-0.483686111690123,0.));
#8103=DIRECTION('center_axis',(0.,0.,1.));
#8104=DIRECTION('ref_axis',(1.,0.,0.));
#8105=DIRECTION('center_axis',(0.,0.,-1.));
#8106=DIRECTION('ref_axis',(-1.,2.01858731750028E-16,0.));
#8107=DIRECTION('center_axis',(0.,1.,0.));
#8108=DIRECTION('ref_axis',(-1.,0.,0.));
#8109=DIRECTION('',(0.,0.,1.));
#8110=DIRECTION('',(-1.,0.,0.));
#8111=DIRECTION('',(0.,0.,1.));
#8112=DIRECTION('center_axis',(-1.,0.,0.));
#8113=DIRECTION('ref_axis',(0.,-1.,0.));
#8114=DIRECTION('',(0.,-1.,0.));
#8115=DIRECTION('center_axis',(1.,0.,0.));
#8116=DIRECTION('ref_axis',(0.,1.,0.));
#8117=DIRECTION('',(0.,0.,1.));
#8118=DIRECTION('',(0.,1.,0.));
#8119=DIRECTION('center_axis',(0.,0.,1.));
#8120=DIRECTION('ref_axis',(1.,0.,0.));
#8121=DIRECTION('',(0.,0.,1.));
#8122=DIRECTION('center_axis',(0.,0.,1.));
#8123=DIRECTION('ref_axis',(1.,0.,0.));
#8124=DIRECTION('center_axis',(0.,0.,1.));
#8125=DIRECTION('ref_axis',(1.,0.,0.));
#8126=DIRECTION('center_axis',(0.,0.,1.));
#8127=DIRECTION('ref_axis',(1.,0.,0.));
#8128=DIRECTION('',(0.,0.,-1.));
#8129=DIRECTION('center_axis',(0.,0.,1.));
#8130=DIRECTION('ref_axis',(1.,0.,0.));
#8131=DIRECTION('',(0.87524153543927,-0.483686111690123,0.));
#8132=DIRECTION('center_axis',(0.,0.,1.));
#8133=DIRECTION('ref_axis',(1.,0.,0.));
#8134=DIRECTION('',(0.87524153543927,-0.483686111690123,0.));
#8135=DIRECTION('',(1.,0.,0.));
#8136=DIRECTION('',(0.,1.,0.));
#8137=DIRECTION('',(-1.,0.,0.));
#8138=DIRECTION('',(-0.694594513699567,0.719401460617409,0.));
#8139=DIRECTION('center_axis',(0.,0.,1.));
#8140=DIRECTION('ref_axis',(1.,0.,0.));
#8141=DIRECTION('',(-0.694594513699567,0.719401460617409,0.));
#8142=DIRECTION('',(-0.447213595499958,-0.894427190999916,0.));
#8143=DIRECTION('center_axis',(0.,0.,1.));
#8144=DIRECTION('ref_axis',(-1.,0.,0.));
#8145=DIRECTION('center_axis',(0.,0.,1.));
#8146=DIRECTION('ref_axis',(1.,0.,0.));
#8147=DIRECTION('center_axis',(0.,-1.,0.));
#8148=DIRECTION('ref_axis',(-1.,0.,0.));
#8149=DIRECTION('center_axis',(0.,0.,1.));
#8150=DIRECTION('ref_axis',(-1.,2.01858731750028E-16,0.));
#8151=DIRECTION('center_axis',(0.,0.,-1.));
#8152=DIRECTION('ref_axis',(1.,0.,0.));
#8153=DIRECTION('center_axis',(0.,0.,-1.));
#8154=DIRECTION('ref_axis',(-1.,0.,0.));
#8155=DIRECTION('center_axis',(0.,0.,-1.));
#8156=DIRECTION('ref_axis',(-1.,0.,0.));
#8157=DIRECTION('',(0.,0.,-1.));
#8158=DIRECTION('center_axis',(0.,0.,-1.));
#8159=DIRECTION('ref_axis',(-1.,0.,0.));
#8160=DIRECTION('center_axis',(0.,-1.,0.));
#8161=DIRECTION('ref_axis',(1.,0.,0.));
#8162=DIRECTION('center_axis',(0.,0.,1.));
#8163=DIRECTION('ref_axis',(1.,0.,0.));
#8164=DIRECTION('',(0.,0.,-1.));
#8165=DIRECTION('',(0.,0.,1.));
#8166=DIRECTION('center_axis',(0.,0.,1.));
#8167=DIRECTION('ref_axis',(-0.483686111690122,-0.87524153543927,0.));
#8168=DIRECTION('',(0.,0.,1.));
#8169=DIRECTION('',(0.,0.,-1.));
#8170=DIRECTION('center_axis',(-0.483686111690123,-0.87524153543927,0.));
#8171=DIRECTION('ref_axis',(0.87524153543927,-0.483686111690123,0.));
#8172=DIRECTION('',(0.,0.,1.));
#8173=DIRECTION('center_axis',(0.719401460617409,0.694594513699567,0.));
#8174=DIRECTION('ref_axis',(-0.694594513699567,0.719401460617409,0.));
#8175=DIRECTION('',(0.,0.,1.));
#8176=DIRECTION('center_axis',(-0.483686111690123,-0.87524153543927,0.));
#8177=DIRECTION('ref_axis',(0.87524153543927,-0.483686111690123,0.));
#8178=DIRECTION('center_axis',(-0.894427190999916,0.447213595499958,0.));
#8179=DIRECTION('ref_axis',(-0.447213595499958,-0.894427190999916,0.));
#8180=DIRECTION('',(0.,0.,1.));
#8181=DIRECTION('center_axis',(0.719401460617409,0.694594513699567,0.));
#8182=DIRECTION('ref_axis',(-0.694594513699567,0.719401460617409,0.));
#8183=DIRECTION('center_axis',(0.,1.,0.));
#8184=DIRECTION('ref_axis',(-1.,0.,0.));
#8185=DIRECTION('',(0.,0.,1.));
#8186=DIRECTION('center_axis',(1.,0.,0.));
#8187=DIRECTION('ref_axis',(0.,1.,0.));
#8188=DIRECTION('',(0.,0.,1.));
#8189=DIRECTION('center_axis',(0.,-1.,0.));
#8190=DIRECTION('ref_axis',(1.,0.,0.));
#9571=CARTESIAN_POINT('',(0.,0.,0.));
#9572=CARTESIAN_POINT('Origin',(6.,-2.5,0.3));
#9573=CARTESIAN_POINT('',(5.83,-2.5,0.6));
#9574=CARTESIAN_POINT('Origin',(6.,-2.5,0.6));
#9575=CARTESIAN_POINT('',(5.83,-2.5,0.));
#9576=CARTESIAN_POINT('',(5.83,-2.5,0.3));
#9577=CARTESIAN_POINT('Origin',(6.,-2.5,0.));
#9578=CARTESIAN_POINT('Origin',(14.,-2.5,0.3));
#9579=CARTESIAN_POINT('',(13.83,-2.5,0.6));
#9580=CARTESIAN_POINT('Origin',(14.,-2.5,0.6));
#9581=CARTESIAN_POINT('',(13.83,-2.5,0.));
#9582=CARTESIAN_POINT('',(13.83,-2.5,0.3));
#9583=CARTESIAN_POINT('Origin',(14.,-2.5,0.));
#9584=CARTESIAN_POINT('Origin',(0.,0.,0.3));
#9585=CARTESIAN_POINT('',(-0.41,5.02105187650415E-17,0.6));
#9586=CARTESIAN_POINT('Origin',(0.,0.,0.6));
#9587=CARTESIAN_POINT('',(-0.41,5.02105187650415E-17,0.));
#9588=CARTESIAN_POINT('',(-0.41,5.02105187650415E-17,0.3));
#9589=CARTESIAN_POINT('Origin',(0.,0.,0.));
#9590=CARTESIAN_POINT('Origin',(-2.2,-0.025,-0.625));
#9591=CARTESIAN_POINT('',(-2.2,0.2,-0.5));
#9592=CARTESIAN_POINT('',(-2.2,-0.2,-0.5));
#9593=CARTESIAN_POINT('',(-2.2,0.2375,-0.5));
#9594=CARTESIAN_POINT('',(-2.2,-0.2,-0.8));
#9595=CARTESIAN_POINT('',(-2.2,-0.2,-0.8));
#9596=CARTESIAN_POINT('',(-2.2,-0.2,-0.8));
#9597=CARTESIAN_POINT('Origin',(-6.8,-0.2,-0.8));
#9598=CARTESIAN_POINT('',(-6.8,-0.2,-0.8));
#9599=CARTESIAN_POINT('',(-6.8,0.199999999999998,-0.5));
#9600=CARTESIAN_POINT('',(-6.8,-0.2,-0.8));
#9601=CARTESIAN_POINT('',(-2.2,-0.2,-0.8));
#9602=CARTESIAN_POINT('',(-5.55,0.2,-0.5));
#9603=CARTESIAN_POINT('Origin',(-6.8,-0.025,-0.625));
#9604=CARTESIAN_POINT('',(-6.8,-0.2,-0.5));
#9605=CARTESIAN_POINT('',(-6.8,0.2375,-0.5));
#9606=CARTESIAN_POINT('',(-6.8,-0.2,-0.8));
#9607=CARTESIAN_POINT('Origin',(-4.3,0.5,-0.5));
#9608=CARTESIAN_POINT('',(-2.,0.0666666666666669,-0.5));
#9609=CARTESIAN_POINT('',(-1.6,0.6,-0.5));
#9610=CARTESIAN_POINT('',(-2.,1.2,-0.5));
#9611=CARTESIAN_POINT('',(-2.,0.85,-0.5));
#9612=CARTESIAN_POINT('',(-2.4,1.2,-0.5));
#9613=CARTESIAN_POINT('',(-2.4,1.2,-0.5));
#9614=CARTESIAN_POINT('Origin',(-0.70745614035088,-16.4271929824561,-0.5));
#9615=CARTESIAN_POINT('Origin',(-4.3,0.5,-0.5));
#9616=CARTESIAN_POINT('Origin',(-6.8,1.38777878078145E-17,-0.5));
#9617=CARTESIAN_POINT('Origin',(-2.2,-0.2,-0.8));
#9618=CARTESIAN_POINT('',(-2.,0.0666666666666668,-0.8));
#9619=CARTESIAN_POINT('',(-2.,0.0666666666666667,-0.4));
#9620=CARTESIAN_POINT('',(-1.6,0.6,-0.8));
#9621=CARTESIAN_POINT('Origin',(-6.8,1.38777878078145E-17,-0.8));
#9622=CARTESIAN_POINT('',(-6.8,0.199999999999998,-0.8));
#9623=CARTESIAN_POINT('Origin',(-6.8,1.38777878078145E-17,-0.8));
#9624=CARTESIAN_POINT('',(-6.8,0.199999999999998,-0.8));
#9625=CARTESIAN_POINT('Origin',(-0.70745614035088,-16.4271929824561,-0.8));
#9626=CARTESIAN_POINT('',(-2.4,1.2,-0.8));
#9627=CARTESIAN_POINT('Origin',(-0.70745614035088,-16.4271929824561,-0.8));
#9628=CARTESIAN_POINT('',(-2.4,1.2,-0.8));
#9629=CARTESIAN_POINT('Origin',(-1.8,0.6,-0.8));
#9630=CARTESIAN_POINT('',(-1.6,1.2,-0.8));
#9631=CARTESIAN_POINT('',(-1.6,0.,-0.8));
#9632=CARTESIAN_POINT('',(-1.6,1.2,-0.8));
#9633=CARTESIAN_POINT('',(-2.,0.,-0.8));
#9634=CARTESIAN_POINT('',(-1.6,0.,-0.8));
#9635=CARTESIAN_POINT('',(-2.,0.,-0.8));
#9636=CARTESIAN_POINT('',(-2.,1.2,-0.8));
#9637=CARTESIAN_POINT('Origin',(-1.6,0.,-0.8));
#9638=CARTESIAN_POINT('',(-1.6,1.2,0.));
#9639=CARTESIAN_POINT('',(-1.6,1.2,-0.8));
#9640=CARTESIAN_POINT('',(-1.6,0.,0.));
#9641=CARTESIAN_POINT('',(-1.6,0.,0.));
#9642=CARTESIAN_POINT('',(-1.6,0.,-0.8));
#9643=CARTESIAN_POINT('Origin',(-2.,0.,0.));
#9644=CARTESIAN_POINT('',(-1.4,0.,0.));
#9645=CARTESIAN_POINT('',(-1.2,0.,0.));
#9646=CARTESIAN_POINT('',(-1.4,0.,0.6));
#9647=CARTESIAN_POINT('',(-1.4,0.,0.));
#9648=CARTESIAN_POINT('',(-2.,0.,0.6));
#9649=CARTESIAN_POINT('',(-1.2,0.,0.6));
#9650=CARTESIAN_POINT('',(-2.,0.,0.));
#9651=CARTESIAN_POINT('Origin',(0.,0.,0.));
#9652=CARTESIAN_POINT('',(-1.2,1.2,0.));
#9653=CARTESIAN_POINT('',(-2.,1.2,0.));
#9654=CARTESIAN_POINT('',(-1.2,0.721110255092798,0.));
#9655=CARTESIAN_POINT('',(-1.2,1.2,0.));
#9656=CARTESIAN_POINT('',(0.993295878967653,0.986591757935306,0.));
#9657=CARTESIAN_POINT('Origin',(0.,0.,0.));
#9658=CARTESIAN_POINT('',(1.,1.,0.));
#9659=CARTESIAN_POINT('',(1.,1.,0.));
#9660=CARTESIAN_POINT('',(2.26270761578574,-0.307804316349519,0.));
#9661=CARTESIAN_POINT('',(3.8,-1.9,0.));
#9662=CARTESIAN_POINT('',(3.79686161498349,-1.89674952980433,0.));
#9663=CARTESIAN_POINT('Origin',(2.1,-2.,0.));
#9664=CARTESIAN_POINT('',(3.8,-1.9,0.));
#9665=CARTESIAN_POINT('',(3.8,-1.9,0.));
#9666=CARTESIAN_POINT('',(15.2,-1.9,0.));
#9667=CARTESIAN_POINT('',(15.2,-1.9,0.));
#9668=CARTESIAN_POINT('',(15.2,-3.1,0.));
#9669=CARTESIAN_POINT('',(15.2,-3.1,0.));
#9670=CARTESIAN_POINT('',(3.8,-3.1,0.));
#9671=CARTESIAN_POINT('',(3.8,-3.1,0.));
#9672=CARTESIAN_POINT('',(3.51486278039743,-2.94242416811437,0.));
#9673=CARTESIAN_POINT('',(0.,-1.,0.));
#9674=CARTESIAN_POINT('',(0.549222100239177,-1.30351747644797,0.));
#9675=CARTESIAN_POINT('Origin',(2.1,-2.,0.));
#9676=CARTESIAN_POINT('',(0.533017816115691,-1.29456247732709,0.));
#9677=CARTESIAN_POINT('',(0.,-1.,0.));
#9678=CARTESIAN_POINT('Origin',(0.,0.,0.));
#9679=CARTESIAN_POINT('',(0.9,-2.,0.));
#9680=CARTESIAN_POINT('Origin',(2.1,-2.,0.));
#9681=CARTESIAN_POINT('Origin',(-1.2,1.2,0.));
#9682=CARTESIAN_POINT('',(-2.,1.2,0.6));
#9683=CARTESIAN_POINT('',(-2.,1.2,0.));
#9684=CARTESIAN_POINT('',(-1.2,1.2,0.6));
#9685=CARTESIAN_POINT('',(-2.,1.2,0.6));
#9686=CARTESIAN_POINT('',(-1.2,1.2,0.));
#9687=CARTESIAN_POINT('Origin',(-2.,1.2,0.));
#9688=CARTESIAN_POINT('',(-2.,0.,0.6));
#9689=CARTESIAN_POINT('Origin',(-1.2,0.,0.));
#9690=CARTESIAN_POINT('',(-1.2,0.721110255092798,0.6));
#9691=CARTESIAN_POINT('',(-1.2,0.721110255092798,0.));
#9692=CARTESIAN_POINT('',(-1.2,1.2,0.6));
#9693=CARTESIAN_POINT('Origin',(0.,0.,0.));
#9694=CARTESIAN_POINT('',(0.533017816115691,-1.29456247732709,0.6));
#9695=CARTESIAN_POINT('',(0.533017816115691,-1.29456247732709,0.));
#9696=CARTESIAN_POINT('Origin',(0.,0.,0.6));
#9697=CARTESIAN_POINT('Origin',(0.,0.,0.));
#9698=CARTESIAN_POINT('',(0.993295878967653,0.986591757935306,0.6));
#9699=CARTESIAN_POINT('Origin',(0.,0.,0.6));
#9700=CARTESIAN_POINT('',(0.993295878967653,0.986591757935306,0.));
#9701=CARTESIAN_POINT('Origin',(0.,0.,0.6));
#9702=CARTESIAN_POINT('',(0.549222100239177,-1.30351747644797,0.6));
#9703=CARTESIAN_POINT('',(0.,-1.,0.6));
#9704=CARTESIAN_POINT('',(3.51486278039743,-2.94242416811437,0.6));
#9705=CARTESIAN_POINT('Origin',(2.1,-2.,0.6));
#9706=CARTESIAN_POINT('',(3.8,-3.1,0.6));
#9707=CARTESIAN_POINT('',(0.,-1.,0.6));
#9708=CARTESIAN_POINT('',(15.2,-3.1,0.6));
#9709=CARTESIAN_POINT('',(3.8,-3.1,0.6));
#9710=CARTESIAN_POINT('',(15.2,-1.9,0.6));
#9711=CARTESIAN_POINT('',(15.2,-3.1,0.6));
#9712=CARTESIAN_POINT('',(3.8,-1.9,0.6));
#9713=CARTESIAN_POINT('',(15.2,-1.9,0.6));
#9714=CARTESIAN_POINT('',(3.79686161498349,-1.89674952980433,0.6));
#9715=CARTESIAN_POINT('',(3.8,-1.9,0.6));
#9716=CARTESIAN_POINT('',(2.26270761578574,-0.307804316349519,0.6));
#9717=CARTESIAN_POINT('Origin',(2.1,-2.,0.6));
#9718=CARTESIAN_POINT('',(1.,1.,0.6));
#9719=CARTESIAN_POINT('',(3.8,-1.9,0.6));
#9720=CARTESIAN_POINT('',(1.,1.,0.6));
#9721=CARTESIAN_POINT('',(3.3,-2.,0.6));
#9722=CARTESIAN_POINT('Origin',(2.1,-2.,0.6));
#9723=CARTESIAN_POINT('Origin',(2.1,-2.,0.1));
#9724=CARTESIAN_POINT('',(1.,-2.,0.1));
#9725=CARTESIAN_POINT('Origin',(0.9,-2.,0.1));
#9726=CARTESIAN_POINT('Origin',(2.1,-2.,0.1));
#9727=CARTESIAN_POINT('Origin',(2.1,-2.,0.3));
#9728=CARTESIAN_POINT('',(3.2,-2.,0.5));
#9729=CARTESIAN_POINT('',(1.,-2.,0.5));
#9730=CARTESIAN_POINT('Origin',(2.1,-2.,0.5));
#9731=CARTESIAN_POINT('Origin',(2.1,-2.,0.5));
#9732=CARTESIAN_POINT('',(1.,-2.,0.3));
#9733=CARTESIAN_POINT('Origin',(2.1,-2.,0.5));
#9734=CARTESIAN_POINT('Origin',(3.3,-2.,0.5));
#9735=CARTESIAN_POINT('Origin',(2.1,-2.,0.));
#9736=CARTESIAN_POINT('',(2.26270761578574,-0.307804316349519,0.));
#9737=CARTESIAN_POINT('',(3.79686161498349,-1.89674952980433,0.));
#9738=CARTESIAN_POINT('Origin',(2.1,-2.,0.));
#9739=CARTESIAN_POINT('',(0.549222100239177,-1.30351747644797,0.));
#9740=CARTESIAN_POINT('',(3.51486278039743,-2.94242416811437,0.));
#9741=CARTESIAN_POINT('Origin',(0.,-1.,0.));
#9742=CARTESIAN_POINT('',(3.8,-3.1,0.));
#9743=CARTESIAN_POINT('Origin',(3.8,-1.9,0.));
#9744=CARTESIAN_POINT('',(3.8,-1.9,0.));
#9745=CARTESIAN_POINT('Origin',(0.,-1.,0.));
#9746=CARTESIAN_POINT('Origin',(1.,1.,0.));
#9747=CARTESIAN_POINT('',(1.,1.,0.));
#9748=CARTESIAN_POINT('Origin',(3.8,-1.9,0.));
#9749=CARTESIAN_POINT('Origin',(15.2,-1.9,0.));
#9750=CARTESIAN_POINT('',(15.2,-1.9,0.));
#9751=CARTESIAN_POINT('Origin',(15.2,-3.1,0.));
#9752=CARTESIAN_POINT('',(15.2,-3.1,0.));
#9753=CARTESIAN_POINT('Origin',(3.8,-3.1,0.));
#19448=UNCERTAINTY_MEASURE_WITH_UNIT(LENGTH_MEASURE(0.001),#19472,
'DISTANCE_ACCURACY_VALUE',
'Maximum model space distance between geometric entities at asserted c
onnectivities');
#19458=UNCERTAINTY_MEASURE_WITH_UNIT(LENGTH_MEASURE(0.001),#19472,
'DISTANCE_ACCURACY_VALUE',
'Maximum model space distance between geometric entities at asserted c
onnectivities');
#19461=(
GEOMETRIC_REPRESENTATION_CONTEXT(3)
GLOBAL_UNCERTAINTY_ASSIGNED_CONTEXT((#19448))
GLOBAL_UNIT_ASSIGNED_CONTEXT((#19472,#19474,#19475))
REPRESENTATION_CONTEXT('','3D')
);
#19471=(
GEOMETRIC_REPRESENTATION_CONTEXT(3)
GLOBAL_UNCERTAINTY_ASSIGNED_CONTEXT((#19458))
GLOBAL_UNIT_ASSIGNED_CONTEXT((#19472,#19474,#19475))
REPRESENTATION_CONTEXT('','3D')
);
#19472=(
LENGTH_UNIT()
NAMED_UNIT(*)
SI_UNIT(.CENTI.,.METRE.)
);
#19474=(
NAMED_UNIT(*)
PLANE_ANGLE_UNIT()
SI_UNIT($,.RADIAN.)
);
#19475=(
NAMED_UNIT(*)
SI_UNIT($,.STERADIAN.)
SOLID_ANGLE_UNIT()
);
#19478=SHAPE_DEFINITION_REPRESENTATION(#19490,#19518);
#19490=PRODUCT_DEFINITION_SHAPE('',$,#19531);
#19518=SHAPE_REPRESENTATION('',(#7333),#19461);
#19528=PRODUCT_DEFINITION_CONTEXT('part definition',#19566,'design');
#19531=PRODUCT_DEFINITION('Moving jaw and handle',
'Moving jaw and handle',#19543,#19528);
#19543=PRODUCT_DEFINITION_FORMATION('',$,#19570);
#19566=APPLICATION_CONTEXT(
'Core Data for Automotive Mechanical Design Process');
#19567=PRODUCT_CONTEXT('part definition',#19566,'mechanical');
#19570=PRODUCT('Moving jaw and handle','Moving jaw and handle',$,(#19567));
#19581=PRESENTATION_STYLE_ASSIGNMENT((#19589));
#19589=SURFACE_STYLE_USAGE(.BOTH.,#19597);
#19597=SURFACE_SIDE_STYLE('',(#19605));
#19605=SURFACE_STYLE_FILL_AREA(#19613);
#19613=FILL_AREA_STYLE('Tool steel gray',(#19621));
#19621=FILL_AREA_STYLE_COLOUR('Tool steel gray',#19629);
#19629=COLOUR_RGB('Tool steel gray',0.607843137254902,0.643137254901961,
0.698039215686274);
ENDSEC;
END-ISO-10303-21;
